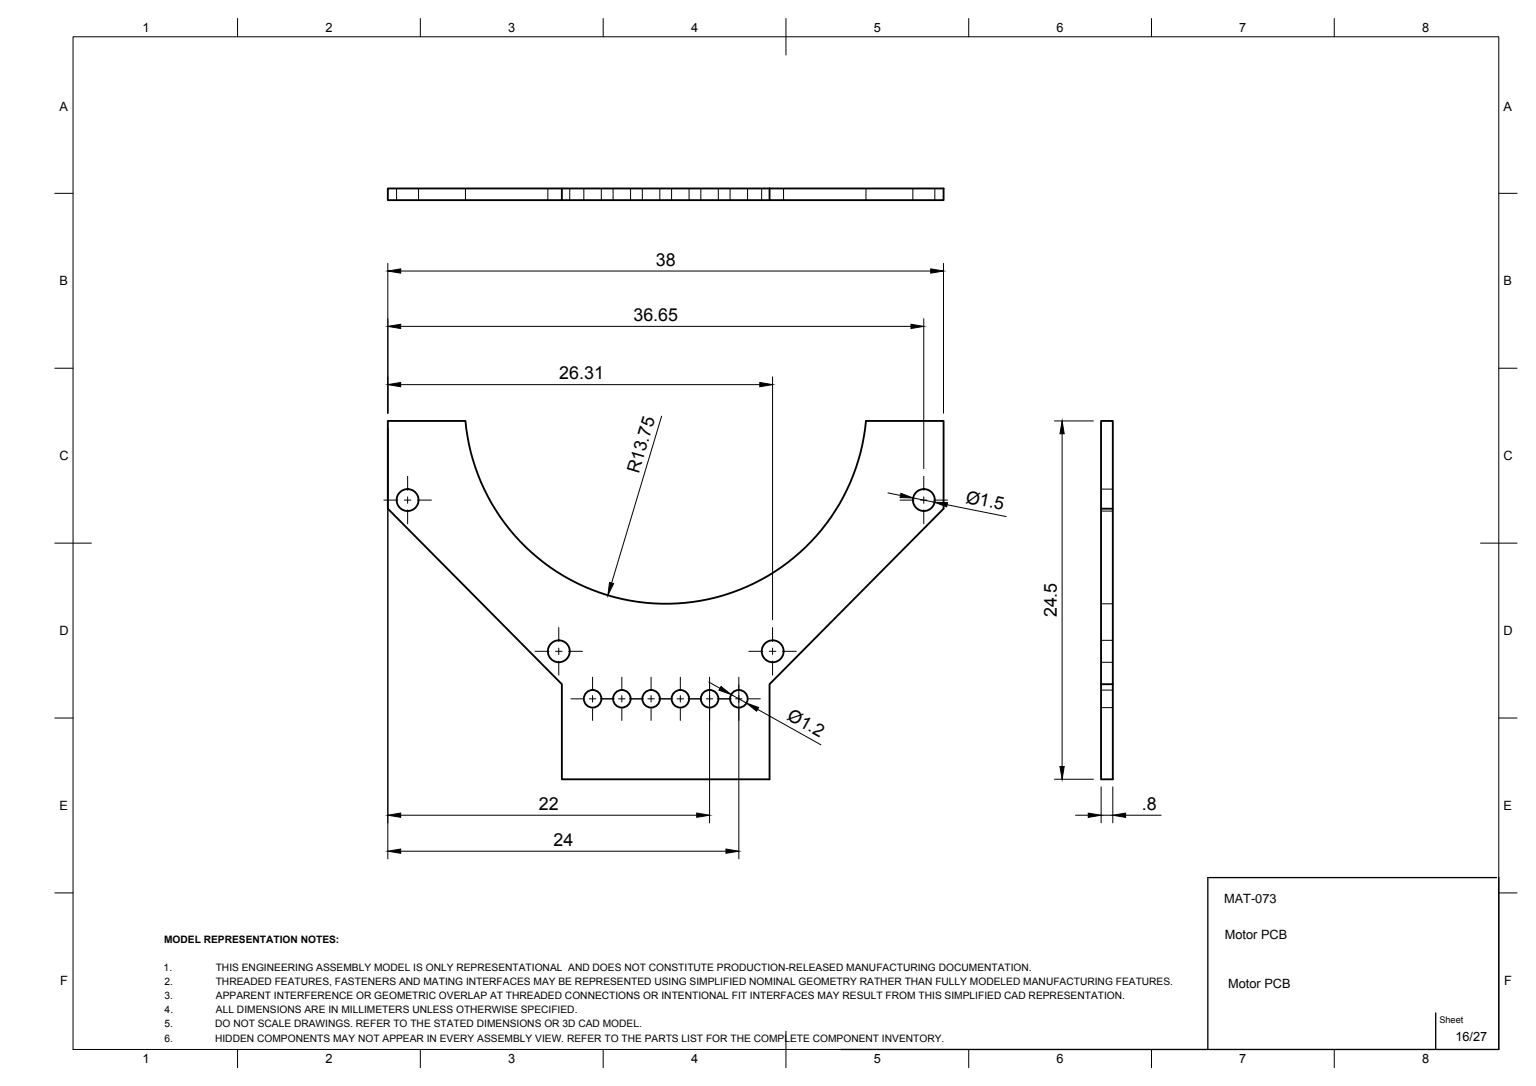
ISO-10303-21;
HEADER;
/* Generated by software containing ST-Developer
 * from STEP Tools, Inc. (www.steptools.com) 
 */

FILE_DESCRIPTION(
/* description */ ('CAx-IF Rec.Pracs.---Representation and Presentation of Product Manufa
cturing Information (PMI)---4.0---2014-10-13'),
/* implementation_level */ '2;1');

FILE_NAME(
/* name */ 'Motor PCB.step',
/* time_stamp */ '2026-10-24T18:52:33-07:00',
/* author */ (''),
/* organization */ (''),
/* preprocessor_version */ 'ST-DEVELOPER v20.2',
/* originating_system */ 'Autodesk Translation Framework v15.17.0.0',
/* authorisation */ '');

FILE_SCHEMA (('AP242_MANAGED_MODEL_BASED_3D_ENGINEERING_MIM_LF { 1 0 10303 442 2 1 4 }'));
ENDSEC;

DATA;
#10=MECHANICAL_DESIGN_GEOMETRIC_PRESENTATION_REPRESENTATION('',(#429),#34876);
#363=SHAPE_REPRESENTATION_RELATIONSHIP('SRR','None',#35000,#396);
#396=ADVANCED_BREP_SHAPE_REPRESENTATION('',(#462),#34858);
#429=STYLED_ITEM('',(#35161),#462);
#462=MANIFOLD_SOLID_BREP('Motor PCB',#19569);
#536=FACE_BOUND('',#6495,.T.);
#537=FACE_BOUND('',#6496,.T.);
#538=FACE_BOUND('',#6497,.T.);
#539=FACE_BOUND('',#6498,.T.);
#540=FACE_BOUND('',#6499,.T.);
#541=FACE_BOUND('',#6500,.T.);
#542=FACE_BOUND('',#6501,.T.);
#543=FACE_BOUND('',#6502,.T.);
#544=FACE_BOUND('',#6503,.T.);
#545=FACE_BOUND('',#6504,.T.);
#546=FACE_BOUND('',#6506,.T.);
#547=FACE_BOUND('',#6507,.T.);
#548=FACE_BOUND('',#6508,.T.);
#549=FACE_BOUND('',#6509,.T.);
#550=FACE_BOUND('',#6510,.T.);
#551=FACE_BOUND('',#6511,.T.);
#552=FACE_BOUND('',#6512,.T.);
#553=FACE_BOUND('',#6513,.T.);
#554=FACE_BOUND('',#6514,.T.);
#555=FACE_BOUND('',#6515,.T.);
#882=PLANE('',#21246);
#883=PLANE('',#21247);
#884=PLANE('',#21248);
#885=PLANE('',#21249);
#886=PLANE('',#21250);
#887=PLANE('',#21251);
#888=PLANE('',#21252);
#889=PLANE('',#21256);
#890=PLANE('',#21257);
#891=PLANE('',#21258);
#892=PLANE('',#21259);
#1947=LINE('',#31950,#3546);
#1948=LINE('',#31956,#3547);
#1949=LINE('',#31962,#3548);
#1950=LINE('',#31968,#3549);
#1951=LINE('',#31974,#3550);
#1952=LINE('',#31980,#3551);
#1953=LINE('',#31986,#3552);
#1954=LINE('',#31992,#3553);
#1955=LINE('',#31998,#3554);
#1956=LINE('',#32004,#3555);
#1957=LINE('',#32009,#3556);
#1958=LINE('',#32011,#3557);
#1959=LINE('',#32013,#3558);
#1960=LINE('',#32014,#3559);
#1961=LINE('',#32017,#3560);
#1962=LINE('',#32019,#3561);
#1963=LINE('',#32020,#3562);
#1964=LINE('',#32024,#3563);
#1965=LINE('',#32026,#3564);
#1966=LINE('',#32028,#3565);
#1967=LINE('',#32029,#3566);
#1968=LINE('',#32031,#3567);
#1969=LINE('',#32032,#3568);
#1970=LINE('',#32036,#3569);
#1971=LINE('',#32038,#3570);
#1972=LINE('',#32040,#3571);
#1973=LINE('',#32041,#3572);
#1974=LINE('',#32044,#3573);
#1975=LINE('',#32046,#3574);
#1976=LINE('',#32047,#3575);
#1977=LINE('',#32049,#3576);
#1978=LINE('',#32050,#3577);
#1979=LINE('',#32056,#3578);
#1980=LINE('',#32059,#3579);
#1981=LINE('',#32061,#3580);
#1982=LINE('',#32062,#3581);
#1983=LINE('',#32064,#3582);
#1984=LINE('',#32065,#3583);
#3546=VECTOR('',#25656,0.00075);
#3547=VECTOR('',#25663,0.00075);
#3548=VECTOR('',#25670,0.00075);
#3549=VECTOR('',#25677,0.00075);
#3550=VECTOR('',#25684,0.0006);
#3551=VECTOR('',#25691,0.0006);
#3552=VECTOR('',#25698,0.0006);
#3553=VECTOR('',#25705,0.0006);
#3554=VECTOR('',#25712,0.0006);
#3555=VECTOR('',#25719,0.0006);
#3556=VECTOR('',#25724,1.);
#3557=VECTOR('',#25725,1.);
#3558=VECTOR('',#25726,1.);
#3559=VECTOR('',#25727,1.);
#3560=VECTOR('',#25730,1.);
#3561=VECTOR('',#25731,1.);
#3562=VECTOR('',#25732,1.);
#3563=VECTOR('',#25735,1.);
#3564=VECTOR('',#25736,1.);
#3565=VECTOR('',#25737,1.);
#3566=VECTOR('',#25738,1.);
#3567=VECTOR('',#25741,1.);
#3568=VECTOR('',#25742,1.);
#3569=VECTOR('',#25745,1.);
#3570=VECTOR('',#25746,1.);
#3571=VECTOR('',#25747,1.);
#3572=VECTOR('',#25748,1.);
#3573=VECTOR('',#25751,1.);
#3574=VECTOR('',#25752,1.);
#3575=VECTOR('',#25753,1.);
#3576=VECTOR('',#25756,1.);
#3577=VECTOR('',#25757,1.);
#3578=VECTOR('',#25764,1.);
#3579=VECTOR('',#25767,1.);
#3580=VECTOR('',#25768,1.);
#3581=VECTOR('',#25769,1.);
#3582=VECTOR('',#25772,1.);
#3583=VECTOR('',#25773,1.);
#4551=CYLINDRICAL_SURFACE('',#21216,0.00075);
#4552=CYLINDRICAL_SURFACE('',#21219,0.00075);
#4553=CYLINDRICAL_SURFACE('',#21222,0.00075);
#4554=CYLINDRICAL_SURFACE('',#21225,0.00075);
#4555=CYLINDRICAL_SURFACE('',#21228,0.0006);
#4556=CYLINDRICAL_SURFACE('',#21231,0.0006);
#4557=CYLINDRICAL_SURFACE('',#21234,0.0006);
#4558=CYLINDRICAL_SURFACE('',#21237,0.0006);
#4559=CYLINDRICAL_SURFACE('',#21240,0.0006);
#4560=CYLINDRICAL_SURFACE('',#21243,0.0006);
#4561=CYLINDRICAL_SURFACE('',#21253,0.01375);
#5373=FACE_OUTER_BOUND('',#6474,.T.);
#5374=FACE_OUTER_BOUND('',#6475,.T.);
#5375=FACE_OUTER_BOUND('',#6476,.T.);
#5376=FACE_OUTER_BOUND('',#6477,.T.);
#5377=FACE_OUTER_BOUND('',#6478,.T.);
#5378=FACE_OUTER_BOUND('',#6479,.T.);
#5379=FACE_OUTER_BOUND('',#6480,.T.);
#5380=FACE_OUTER_BOUND('',#6481,.T.);
#5381=FACE_OUTER_BOUND('',#6482,.T.);
#5382=FACE_OUTER_BOUND('',#6483,.T.);
#5383=FACE_OUTER_BOUND('',#6484,.T.);
#5384=FACE_OUTER_BOUND('',#6485,.T.);
#5385=FACE_OUTER_BOUND('',#6486,.T.);
#5386=FACE_OUTER_BOUND('',#6487,.T.);
#5387=FACE_OUTER_BOUND('',#6488,.T.);
#5388=FACE_OUTER_BOUND('',#6489,.T.);
#5389=FACE_OUTER_BOUND('',#6490,.T.);
#5390=FACE_OUTER_BOUND('',#6491,.T.);
#5391=FACE_OUTER_BOUND('',#6492,.T.);
#5392=FACE_OUTER_BOUND('',#6493,.T.);
#5393=FACE_OUTER_BOUND('',#6494,.T.);
#5394=FACE_OUTER_BOUND('',#6505,.T.);
#6474=EDGE_LOOP('',(#15914,#15915,#15916,#15917));
#6475=EDGE_LOOP('',(#15918,#15919,#15920,#15921));
#6476=EDGE_LOOP('',(#15922,#15923,#15924,#15925));
#6477=EDGE_LOOP('',(#15926,#15927,#15928,#15929));
#6478=EDGE_LOOP('',(#15930,#15931,#15932,#15933));
#6479=EDGE_LOOP('',(#15934,#15935,#15936,#15937));
#6480=EDGE_LOOP('',(#15938,#15939,#15940,#15941));
#6481=EDGE_LOOP('',(#15942,#15943,#15944,#15945));
#6482=EDGE_LOOP('',(#15946,#15947,#15948,#15949));
#6483=EDGE_LOOP('',(#15950,#15951,#15952,#15953));
#6484=EDGE_LOOP('',(#15954,#15955,#15956,#15957));
#6485=EDGE_LOOP('',(#15958,#15959,#15960,#15961));
#6486=EDGE_LOOP('',(#15962,#15963,#15964,#15965));
#6487=EDGE_LOOP('',(#15966,#15967,#15968,#15969));
#6488=EDGE_LOOP('',(#15970,#15971,#15972,#15973));
#6489=EDGE_LOOP('',(#15974,#15975,#15976,#15977));
#6490=EDGE_LOOP('',(#15978,#15979,#15980,#15981));
#6491=EDGE_LOOP('',(#15982,#15983,#15984,#15985));
#6492=EDGE_LOOP('',(#15986,#15987,#15988,#15989));
#6493=EDGE_LOOP('',(#15990,#15991,#15992,#15993));
#6494=EDGE_LOOP('',(#15994,#15995,#15996,#15997,#15998,#15999,#16000,#16001,
#16002,#16003));
#6495=EDGE_LOOP('',(#16004));
#6496=EDGE_LOOP('',(#16005));
#6497=EDGE_LOOP('',(#16006));
#6498=EDGE_LOOP('',(#16007));
#6499=EDGE_LOOP('',(#16008));
#6500=EDGE_LOOP('',(#16009));
#6501=EDGE_LOOP('',(#16010));
#6502=EDGE_LOOP('',(#16011));
#6503=EDGE_LOOP('',(#16012));
#6504=EDGE_LOOP('',(#16013));
#6505=EDGE_LOOP('',(#16014,#16015,#16016,#16017,#16018,#16019,#16020,#16021,
#16022,#16023));
#6506=EDGE_LOOP('',(#16024));
#6507=EDGE_LOOP('',(#16025));
#6508=EDGE_LOOP('',(#16026));
#6509=EDGE_LOOP('',(#16027));
#6510=EDGE_LOOP('',(#16028));
#6511=EDGE_LOOP('',(#16029));
#6512=EDGE_LOOP('',(#16030));
#6513=EDGE_LOOP('',(#16031));
#6514=EDGE_LOOP('',(#16032));
#6515=EDGE_LOOP('',(#16033));
#7549=CIRCLE('',#21217,0.00075000000001);
#7550=CIRCLE('',#21218,0.00075000000001);
#7551=CIRCLE('',#21220,0.00075000000001);
#7552=CIRCLE('',#21221,0.00075000000001);
#7553=CIRCLE('',#21223,0.00075000000001);
#7554=CIRCLE('',#21224,0.00075000000001);
#7555=CIRCLE('',#21226,0.00075000000001);
#7556=CIRCLE('',#21227,0.00075000000001);
#7557=CIRCLE('',#21229,0.00060000000001);
#7558=CIRCLE('',#21230,0.00060000000001);
#7559=CIRCLE('',#21232,0.00060000000001);
#7560=CIRCLE('',#21233,0.00060000000001);
#7561=CIRCLE('',#21235,0.00060000000001);
#7562=CIRCLE('',#21236,0.00060000000001);
#7563=CIRCLE('',#21238,0.00060000000001);
#7564=CIRCLE('',#21239,0.00060000000001);
#7565=CIRCLE('',#21241,0.00060000000001);
#7566=CIRCLE('',#21242,0.00060000000001);
#7567=CIRCLE('',#21244,0.00060000000001);
#7568=CIRCLE('',#21245,0.00060000000001);
#7569=CIRCLE('',#21254,0.01375000000001);
#7570=CIRCLE('',#21255,0.01375000000001);
#9101=VERTEX_POINT('',#31947);
#9102=VERTEX_POINT('',#31949);
#9103=VERTEX_POINT('',#31953);
#9104=VERTEX_POINT('',#31955);
#9105=VERTEX_POINT('',#31959);
#9106=VERTEX_POINT('',#31961);
#9107=VERTEX_POINT('',#31965);
#9108=VERTEX_POINT('',#31967);
#9109=VERTEX_POINT('',#31971);
#9110=VERTEX_POINT('',#31973);
#9111=VERTEX_POINT('',#31977);
#9112=VERTEX_POINT('',#31979);
#9113=VERTEX_POINT('',#31983);
#9114=VERTEX_POINT('',#31985);
#9115=VERTEX_POINT('',#31989);
#9116=VERTEX_POINT('',#31991);
#9117=VERTEX_POINT('',#31995);
#9118=VERTEX_POINT('',#31997);
#9119=VERTEX_POINT('',#32001);
#9120=VERTEX_POINT('',#32003);
#9121=VERTEX_POINT('',#32007);
#9122=VERTEX_POINT('',#32008);
#9123=VERTEX_POINT('',#32010);
#9124=VERTEX_POINT('',#32012);
#9125=VERTEX_POINT('',#32016);
#9126=VERTEX_POINT('',#32018);
#9127=VERTEX_POINT('',#32022);
#9128=VERTEX_POINT('',#32023);
#9129=VERTEX_POINT('',#32025);
#9130=VERTEX_POINT('',#32027);
#9131=VERTEX_POINT('',#32034);
#9132=VERTEX_POINT('',#32035);
#9133=VERTEX_POINT('',#32037);
#9134=VERTEX_POINT('',#32039);
#9135=VERTEX_POINT('',#32043);
#9136=VERTEX_POINT('',#32045);
#9137=VERTEX_POINT('',#32052);
#9138=VERTEX_POINT('',#32054);
#9139=VERTEX_POINT('',#32058);
#9140=VERTEX_POINT('',#32060);
#11515=EDGE_CURVE('',#9101,#9101,#7549,.T.);
#11516=EDGE_CURVE('',#9101,#9102,#1947,.T.);
#11517=EDGE_CURVE('',#9102,#9102,#7550,.T.);
#11518=EDGE_CURVE('',#9103,#9103,#7551,.T.);
#11519=EDGE_CURVE('',#9103,#9104,#1948,.T.);
#11520=EDGE_CURVE('',#9104,#9104,#7552,.T.);
#11521=EDGE_CURVE('',#9105,#9105,#7553,.T.);
#11522=EDGE_CURVE('',#9105,#9106,#1949,.T.);
#11523=EDGE_CURVE('',#9106,#9106,#7554,.T.);
#11524=EDGE_CURVE('',#9107,#9107,#7555,.T.);
#11525=EDGE_CURVE('',#9107,#9108,#1950,.T.);
#11526=EDGE_CURVE('',#9108,#9108,#7556,.T.);
#11527=EDGE_CURVE('',#9109,#9109,#7557,.T.);
#11528=EDGE_CURVE('',#9109,#9110,#1951,.T.);
#11529=EDGE_CURVE('',#9110,#9110,#7558,.T.);
#11530=EDGE_CURVE('',#9111,#9111,#7559,.T.);
#11531=EDGE_CURVE('',#9111,#9112,#1952,.T.);
#11532=EDGE_CURVE('',#9112,#9112,#7560,.T.);
#11533=EDGE_CURVE('',#9113,#9113,#7561,.T.);
#11534=EDGE_CURVE('',#9113,#9114,#1953,.T.);
#11535=EDGE_CURVE('',#9114,#9114,#7562,.T.);
#11536=EDGE_CURVE('',#9115,#9115,#7563,.T.);
#11537=EDGE_CURVE('',#9115,#9116,#1954,.T.);
#11538=EDGE_CURVE('',#9116,#9116,#7564,.T.);
#11539=EDGE_CURVE('',#9117,#9117,#7565,.T.);
#11540=EDGE_CURVE('',#9117,#9118,#1955,.T.);
#11541=EDGE_CURVE('',#9118,#9118,#7566,.T.);
#11542=EDGE_CURVE('',#9119,#9119,#7567,.T.);
#11543=EDGE_CURVE('',#9119,#9120,#1956,.T.);
#11544=EDGE_CURVE('',#9120,#9120,#7568,.T.);
#11545=EDGE_CURVE('',#9121,#9122,#1957,.T.);
#11546=EDGE_CURVE('',#9121,#9123,#1958,.T.);
#11547=EDGE_CURVE('',#9123,#9124,#1959,.T.);
#11548=EDGE_CURVE('',#9122,#9124,#1960,.T.);
#11549=EDGE_CURVE('',#9125,#9121,#1961,.T.);
#11550=EDGE_CURVE('',#9125,#9126,#1962,.T.);
#11551=EDGE_CURVE('',#9126,#9123,#1963,.T.);
#11552=EDGE_CURVE('',#9127,#9128,#1964,.T.);
#11553=EDGE_CURVE('',#9127,#9129,#1965,.T.);
#11554=EDGE_CURVE('',#9129,#9130,#1966,.T.);
#11555=EDGE_CURVE('',#9128,#9130,#1967,.T.);
#11556=EDGE_CURVE('',#9122,#9127,#1968,.T.);
#11557=EDGE_CURVE('',#9124,#9129,#1969,.T.);
#11558=EDGE_CURVE('',#9131,#9132,#1970,.T.);
#11559=EDGE_CURVE('',#9132,#9133,#1971,.T.);
#11560=EDGE_CURVE('',#9134,#9133,#1972,.T.);
#11561=EDGE_CURVE('',#9131,#9134,#1973,.T.);
#11562=EDGE_CURVE('',#9135,#9131,#1974,.T.);
#11563=EDGE_CURVE('',#9136,#9134,#1975,.T.);
#11564=EDGE_CURVE('',#9135,#9136,#1976,.T.);
#11565=EDGE_CURVE('',#9135,#9125,#1977,.T.);
#11566=EDGE_CURVE('',#9136,#9126,#1978,.T.);
#11567=EDGE_CURVE('',#9137,#9128,#7569,.T.);
#11568=EDGE_CURVE('',#9138,#9130,#7570,.T.);
#11569=EDGE_CURVE('',#9137,#9138,#1979,.T.);
#11570=EDGE_CURVE('',#9139,#9137,#1980,.T.);
#11571=EDGE_CURVE('',#9140,#9138,#1981,.T.);
#11572=EDGE_CURVE('',#9139,#9140,#1982,.T.);
#11573=EDGE_CURVE('',#9132,#9139,#1983,.T.);
#11574=EDGE_CURVE('',#9133,#9140,#1984,.T.);
#15914=ORIENTED_EDGE('',*,*,#11515,.F.);
#15915=ORIENTED_EDGE('',*,*,#11516,.T.);
#15916=ORIENTED_EDGE('',*,*,#11517,.F.);
#15917=ORIENTED_EDGE('',*,*,#11516,.F.);
#15918=ORIENTED_EDGE('',*,*,#11518,.F.);
#15919=ORIENTED_EDGE('',*,*,#11519,.T.);
#15920=ORIENTED_EDGE('',*,*,#11520,.F.);
#15921=ORIENTED_EDGE('',*,*,#11519,.F.);
#15922=ORIENTED_EDGE('',*,*,#11521,.F.);
#15923=ORIENTED_EDGE('',*,*,#11522,.T.);
#15924=ORIENTED_EDGE('',*,*,#11523,.F.);
#15925=ORIENTED_EDGE('',*,*,#11522,.F.);
#15926=ORIENTED_EDGE('',*,*,#11524,.F.);
#15927=ORIENTED_EDGE('',*,*,#11525,.T.);
#15928=ORIENTED_EDGE('',*,*,#11526,.F.);
#15929=ORIENTED_EDGE('',*,*,#11525,.F.);
#15930=ORIENTED_EDGE('',*,*,#11527,.F.);
#15931=ORIENTED_EDGE('',*,*,#11528,.T.);
#15932=ORIENTED_EDGE('',*,*,#11529,.F.);
#15933=ORIENTED_EDGE('',*,*,#11528,.F.);
#15934=ORIENTED_EDGE('',*,*,#11530,.F.);
#15935=ORIENTED_EDGE('',*,*,#11531,.T.);
#15936=ORIENTED_EDGE('',*,*,#11532,.F.);
#15937=ORIENTED_EDGE('',*,*,#11531,.F.);
#15938=ORIENTED_EDGE('',*,*,#11533,.F.);
#15939=ORIENTED_EDGE('',*,*,#11534,.T.);
#15940=ORIENTED_EDGE('',*,*,#11535,.F.);
#15941=ORIENTED_EDGE('',*,*,#11534,.F.);
#15942=ORIENTED_EDGE('',*,*,#11536,.F.);
#15943=ORIENTED_EDGE('',*,*,#11537,.T.);
#15944=ORIENTED_EDGE('',*,*,#11538,.F.);
#15945=ORIENTED_EDGE('',*,*,#11537,.F.);
#15946=ORIENTED_EDGE('',*,*,#11539,.F.);
#15947=ORIENTED_EDGE('',*,*,#11540,.T.);
#15948=ORIENTED_EDGE('',*,*,#11541,.F.);
#15949=ORIENTED_EDGE('',*,*,#11540,.F.);
#15950=ORIENTED_EDGE('',*,*,#11542,.F.);
#15951=ORIENTED_EDGE('',*,*,#11543,.T.);
#15952=ORIENTED_EDGE('',*,*,#11544,.F.);
#15953=ORIENTED_EDGE('',*,*,#11543,.F.);
#15954=ORIENTED_EDGE('',*,*,#11545,.F.);
#15955=ORIENTED_EDGE('',*,*,#11546,.T.);
#15956=ORIENTED_EDGE('',*,*,#11547,.T.);
#15957=ORIENTED_EDGE('',*,*,#11548,.F.);
#15958=ORIENTED_EDGE('',*,*,#11549,.F.);
#15959=ORIENTED_EDGE('',*,*,#11550,.T.);
#15960=ORIENTED_EDGE('',*,*,#11551,.T.);
#15961=ORIENTED_EDGE('',*,*,#11546,.F.);
#15962=ORIENTED_EDGE('',*,*,#11552,.F.);
#15963=ORIENTED_EDGE('',*,*,#11553,.T.);
#15964=ORIENTED_EDGE('',*,*,#11554,.T.);
#15965=ORIENTED_EDGE('',*,*,#11555,.F.);
#15966=ORIENTED_EDGE('',*,*,#11556,.F.);
#15967=ORIENTED_EDGE('',*,*,#11548,.T.);
#15968=ORIENTED_EDGE('',*,*,#11557,.T.);
#15969=ORIENTED_EDGE('',*,*,#11553,.F.);
#15970=ORIENTED_EDGE('',*,*,#11558,.T.);
#15971=ORIENTED_EDGE('',*,*,#11559,.T.);
#15972=ORIENTED_EDGE('',*,*,#11560,.F.);
#15973=ORIENTED_EDGE('',*,*,#11561,.F.);
#15974=ORIENTED_EDGE('',*,*,#11562,.T.);
#15975=ORIENTED_EDGE('',*,*,#11561,.T.);
#15976=ORIENTED_EDGE('',*,*,#11563,.F.);
#15977=ORIENTED_EDGE('',*,*,#11564,.F.);
#15978=ORIENTED_EDGE('',*,*,#11565,.F.);
#15979=ORIENTED_EDGE('',*,*,#11564,.T.);
#15980=ORIENTED_EDGE('',*,*,#11566,.T.);
#15981=ORIENTED_EDGE('',*,*,#11550,.F.);
#15982=ORIENTED_EDGE('',*,*,#11567,.T.);
#15983=ORIENTED_EDGE('',*,*,#11555,.T.);
#15984=ORIENTED_EDGE('',*,*,#11568,.F.);
#15985=ORIENTED_EDGE('',*,*,#11569,.F.);
#15986=ORIENTED_EDGE('',*,*,#11570,.T.);
#15987=ORIENTED_EDGE('',*,*,#11569,.T.);
#15988=ORIENTED_EDGE('',*,*,#11571,.F.);
#15989=ORIENTED_EDGE('',*,*,#11572,.F.);
#15990=ORIENTED_EDGE('',*,*,#11573,.T.);
#15991=ORIENTED_EDGE('',*,*,#11572,.T.);
#15992=ORIENTED_EDGE('',*,*,#11574,.F.);
#15993=ORIENTED_EDGE('',*,*,#11559,.F.);
#15994=ORIENTED_EDGE('',*,*,#11574,.T.);
#15995=ORIENTED_EDGE('',*,*,#11571,.T.);
#15996=ORIENTED_EDGE('',*,*,#11568,.T.);
#15997=ORIENTED_EDGE('',*,*,#11554,.F.);
#15998=ORIENTED_EDGE('',*,*,#11557,.F.);
#15999=ORIENTED_EDGE('',*,*,#11547,.F.);
#16000=ORIENTED_EDGE('',*,*,#11551,.F.);
#16001=ORIENTED_EDGE('',*,*,#11566,.F.);
#16002=ORIENTED_EDGE('',*,*,#11563,.T.);
#16003=ORIENTED_EDGE('',*,*,#11560,.T.);
#16004=ORIENTED_EDGE('',*,*,#11517,.T.);
#16005=ORIENTED_EDGE('',*,*,#11520,.T.);
#16006=ORIENTED_EDGE('',*,*,#11523,.T.);
#16007=ORIENTED_EDGE('',*,*,#11526,.T.);
#16008=ORIENTED_EDGE('',*,*,#11529,.T.);
#16009=ORIENTED_EDGE('',*,*,#11532,.T.);
#16010=ORIENTED_EDGE('',*,*,#11535,.T.);
#16011=ORIENTED_EDGE('',*,*,#11538,.T.);
#16012=ORIENTED_EDGE('',*,*,#11541,.T.);
#16013=ORIENTED_EDGE('',*,*,#11544,.T.);
#16014=ORIENTED_EDGE('',*,*,#11573,.F.);
#16015=ORIENTED_EDGE('',*,*,#11558,.F.);
#16016=ORIENTED_EDGE('',*,*,#11562,.F.);
#16017=ORIENTED_EDGE('',*,*,#11565,.T.);
#16018=ORIENTED_EDGE('',*,*,#11549,.T.);
#16019=ORIENTED_EDGE('',*,*,#11545,.T.);
#16020=ORIENTED_EDGE('',*,*,#11556,.T.);
#16021=ORIENTED_EDGE('',*,*,#11552,.T.);
#16022=ORIENTED_EDGE('',*,*,#11567,.F.);
#16023=ORIENTED_EDGE('',*,*,#11570,.F.);
#16024=ORIENTED_EDGE('',*,*,#11515,.T.);
#16025=ORIENTED_EDGE('',*,*,#11518,.T.);
#16026=ORIENTED_EDGE('',*,*,#11521,.T.);
#16027=ORIENTED_EDGE('',*,*,#11524,.T.);
#16028=ORIENTED_EDGE('',*,*,#11527,.T.);
#16029=ORIENTED_EDGE('',*,*,#11530,.T.);
#16030=ORIENTED_EDGE('',*,*,#11533,.T.);
#16031=ORIENTED_EDGE('',*,*,#11536,.T.);
#16032=ORIENTED_EDGE('',*,*,#11539,.T.);
#16033=ORIENTED_EDGE('',*,*,#11542,.T.);
#19089=ADVANCED_FACE('',(#5373),#4551,.F.);
#19090=ADVANCED_FACE('',(#5374),#4552,.F.);
#19091=ADVANCED_FACE('',(#5375),#4553,.F.);
#19092=ADVANCED_FACE('',(#5376),#4554,.F.);
#19093=ADVANCED_FACE('',(#5377),#4555,.F.);
#19094=ADVANCED_FACE('',(#5378),#4556,.F.);
#19095=ADVANCED_FACE('',(#5379),#4557,.F.);
#19096=ADVANCED_FACE('',(#5380),#4558,.F.);
#19097=ADVANCED_FACE('',(#5381),#4559,.F.);
#19098=ADVANCED_FACE('',(#5382),#4560,.F.);
#19099=ADVANCED_FACE('',(#5383),#882,.F.);
#19100=ADVANCED_FACE('',(#5384),#883,.F.);
#19101=ADVANCED_FACE('',(#5385),#884,.F.);
#19102=ADVANCED_FACE('',(#5386),#885,.F.);
#19103=ADVANCED_FACE('',(#5387),#886,.T.);
#19104=ADVANCED_FACE('',(#5388),#887,.T.);
#19105=ADVANCED_FACE('',(#5389),#888,.T.);
#19106=ADVANCED_FACE('',(#5390),#4561,.F.);
#19107=ADVANCED_FACE('',(#5391),#889,.T.);
#19108=ADVANCED_FACE('',(#5392),#890,.T.);
#19109=ADVANCED_FACE('',(#5393,#536,#537,#538,#539,#540,#541,#542,#543,
#544,#545),#891,.T.);
#19110=ADVANCED_FACE('',(#5394,#546,#547,#548,#549,#550,#551,#552,#553,
#554,#555),#892,.F.);
#19569=CLOSED_SHELL('',(#19089,#19090,#19091,#19092,#19093,#19094,#19095,
#19096,#19097,#19098,#19099,#19100,#19101,#19102,#19103,#19104,#19105,#19106,
#19107,#19108,#19109,#19110));
#21215=AXIS2_PLACEMENT_3D('',#31945,#25650,#25651);
#21216=AXIS2_PLACEMENT_3D('',#31946,#25652,#25653);
#21217=AXIS2_PLACEMENT_3D('',#31948,#25654,#25655);
#21218=AXIS2_PLACEMENT_3D('',#31951,#25657,#25658);
#21219=AXIS2_PLACEMENT_3D('',#31952,#25659,#25660);
#21220=AXIS2_PLACEMENT_3D('',#31954,#25661,#25662);
#21221=AXIS2_PLACEMENT_3D('',#31957,#25664,#25665);
#21222=AXIS2_PLACEMENT_3D('',#31958,#25666,#25667);
#21223=AXIS2_PLACEMENT_3D('',#31960,#25668,#25669);
#21224=AXIS2_PLACEMENT_3D('',#31963,#25671,#25672);
#21225=AXIS2_PLACEMENT_3D('',#31964,#25673,#25674);
#21226=AXIS2_PLACEMENT_3D('',#31966,#25675,#25676);
#21227=AXIS2_PLACEMENT_3D('',#31969,#25678,#25679);
#21228=AXIS2_PLACEMENT_3D('',#31970,#25680,#25681);
#21229=AXIS2_PLACEMENT_3D('',#31972,#25682,#25683);
#21230=AXIS2_PLACEMENT_3D('',#31975,#25685,#25686);
#21231=AXIS2_PLACEMENT_3D('',#31976,#25687,#25688);
#21232=AXIS2_PLACEMENT_3D('',#31978,#25689,#25690);
#21233=AXIS2_PLACEMENT_3D('',#31981,#25692,#25693);
#21234=AXIS2_PLACEMENT_3D('',#31982,#25694,#25695);
#21235=AXIS2_PLACEMENT_3D('',#31984,#25696,#25697);
#21236=AXIS2_PLACEMENT_3D('',#31987,#25699,#25700);
#21237=AXIS2_PLACEMENT_3D('',#31988,#25701,#25702);
#21238=AXIS2_PLACEMENT_3D('',#31990,#25703,#25704);
#21239=AXIS2_PLACEMENT_3D('',#31993,#25706,#25707);
#21240=AXIS2_PLACEMENT_3D('',#31994,#25708,#25709);
#21241=AXIS2_PLACEMENT_3D('',#31996,#25710,#25711);
#21242=AXIS2_PLACEMENT_3D('',#31999,#25713,#25714);
#21243=AXIS2_PLACEMENT_3D('',#32000,#25715,#25716);
#21244=AXIS2_PLACEMENT_3D('',#32002,#25717,#25718);
#21245=AXIS2_PLACEMENT_3D('',#32005,#25720,#25721);
#21246=AXIS2_PLACEMENT_3D('',#32006,#25722,#25723);
#21247=AXIS2_PLACEMENT_3D('',#32015,#25728,#25729);
#21248=AXIS2_PLACEMENT_3D('',#32021,#25733,#25734);
#21249=AXIS2_PLACEMENT_3D('',#32030,#25739,#25740);
#21250=AXIS2_PLACEMENT_3D('',#32033,#25743,#25744);
#21251=AXIS2_PLACEMENT_3D('',#32042,#25749,#25750);
#21252=AXIS2_PLACEMENT_3D('',#32048,#25754,#25755);
#21253=AXIS2_PLACEMENT_3D('',#32051,#25758,#25759);
#21254=AXIS2_PLACEMENT_3D('',#32053,#25760,#25761);
#21255=AXIS2_PLACEMENT_3D('',#32055,#25762,#25763);
#21256=AXIS2_PLACEMENT_3D('',#32057,#25765,#25766);
#21257=AXIS2_PLACEMENT_3D('',#32063,#25770,#25771);
#21258=AXIS2_PLACEMENT_3D('',#32066,#25774,#25775);
#21259=AXIS2_PLACEMENT_3D('',#32067,#25776,#25777);
#25650=DIRECTION('axis',(0.,0.,1.));
#25651=DIRECTION('refdir',(1.,0.,0.));
#25652=DIRECTION('center_axis',(4.57029560239561E-17,1.,8.81733986229836E-18));
#25653=DIRECTION('ref_axis',(4.44089209850056E-15,-8.81733986229857E-18,
1.));
#25654=DIRECTION('center_axis',(4.57029560239561E-17,1.,8.81733986229836E-18));
#25655=DIRECTION('ref_axis',(4.44089209850056E-15,-8.81733986229857E-18,
1.));
#25656=DIRECTION('',(4.57029560239561E-17,1.,8.81733986229836E-18));
#25657=DIRECTION('center_axis',(-4.57029560239561E-17,-1.,-8.81733986229836E-18));
#25658=DIRECTION('ref_axis',(4.44089209850056E-15,-8.81733986229857E-18,
1.));
#25659=DIRECTION('center_axis',(4.57029560239561E-17,1.,8.81733986229836E-18));
#25660=DIRECTION('ref_axis',(4.44089209850056E-15,-8.81733986229857E-18,
1.));
#25661=DIRECTION('center_axis',(4.57029560239561E-17,1.,8.81733986229836E-18));
#25662=DIRECTION('ref_axis',(4.44089209850056E-15,-8.81733986229857E-18,
1.));
#25663=DIRECTION('',(4.57029560239561E-17,1.,8.81733986229836E-18));
#25664=DIRECTION('center_axis',(-4.57029560239561E-17,-1.,-8.81733986229836E-18));
#25665=DIRECTION('ref_axis',(4.44089209850056E-15,-8.81733986229857E-18,
1.));
#25666=DIRECTION('center_axis',(4.57029560239561E-17,1.,8.81733986229836E-18));
#25667=DIRECTION('ref_axis',(4.44089209850056E-15,-8.81733986229857E-18,
1.));
#25668=DIRECTION('center_axis',(4.57029560239561E-17,1.,8.81733986229836E-18));
#25669=DIRECTION('ref_axis',(4.44089209850056E-15,-8.81733986229857E-18,
1.));
#25670=DIRECTION('',(4.57029560239561E-17,1.,8.81733986229836E-18));
#25671=DIRECTION('center_axis',(-4.57029560239561E-17,-1.,-8.81733986229836E-18));
#25672=DIRECTION('ref_axis',(4.44089209850056E-15,-8.81733986229857E-18,
1.));
#25673=DIRECTION('center_axis',(4.57029560239561E-17,1.,8.81733986229836E-18));
#25674=DIRECTION('ref_axis',(4.44089209850056E-15,-8.81733986229857E-18,
1.));
#25675=DIRECTION('center_axis',(4.57029560239561E-17,1.,8.81733986229836E-18));
#25676=DIRECTION('ref_axis',(4.44089209850056E-15,-8.81733986229857E-18,
1.));
#25677=DIRECTION('',(4.57029560239561E-17,1.,8.81733986229836E-18));
#25678=DIRECTION('center_axis',(-4.57029560239561E-17,-1.,-8.81733986229836E-18));
#25679=DIRECTION('ref_axis',(4.44089209850056E-15,-8.81733986229857E-18,
1.));
#25680=DIRECTION('center_axis',(4.57029560239561E-17,1.,8.81733986229836E-18));
#25681=DIRECTION('ref_axis',(4.44089209850056E-15,-8.81733986229857E-18,
1.));
#25682=DIRECTION('center_axis',(4.57029560239561E-17,1.,8.81733986229836E-18));
#25683=DIRECTION('ref_axis',(4.44089209850056E-15,-8.81733986229856E-18,
1.));
#25684=DIRECTION('',(4.57029560239561E-17,1.,8.81733986229836E-18));
#25685=DIRECTION('center_axis',(-4.57029560239561E-17,-1.,-8.81733986229836E-18));
#25686=DIRECTION('ref_axis',(4.44089209850056E-15,-8.81733986229856E-18,
1.));
#25687=DIRECTION('center_axis',(4.57029560239561E-17,1.,8.81733986229836E-18));
#25688=DIRECTION('ref_axis',(4.44089209850056E-15,-8.81733986229857E-18,
1.));
#25689=DIRECTION('center_axis',(4.57029560239561E-17,1.,8.81733986229836E-18));
#25690=DIRECTION('ref_axis',(4.44089209850056E-15,-8.81733986229856E-18,
1.));
#25691=DIRECTION('',(4.57029560239561E-17,1.,8.81733986229836E-18));
#25692=DIRECTION('center_axis',(-4.57029560239561E-17,-1.,-8.81733986229836E-18));
#25693=DIRECTION('ref_axis',(4.44089209850056E-15,-8.81733986229856E-18,
1.));
#25694=DIRECTION('center_axis',(4.57029560239561E-17,1.,8.81733986229836E-18));
#25695=DIRECTION('ref_axis',(4.44089209850056E-15,-8.81733986229857E-18,
1.));
#25696=DIRECTION('center_axis',(4.57029560239561E-17,1.,8.81733986229836E-18));
#25697=DIRECTION('ref_axis',(4.44089209850056E-15,-8.81733986229856E-18,
1.));
#25698=DIRECTION('',(4.57029560239561E-17,1.,8.81733986229836E-18));
#25699=DIRECTION('center_axis',(-4.57029560239561E-17,-1.,-8.81733986229836E-18));
#25700=DIRECTION('ref_axis',(4.44089209850056E-15,-8.81733986229856E-18,
1.));
#25701=DIRECTION('center_axis',(4.57029560239561E-17,1.,8.81733986229836E-18));
#25702=DIRECTION('ref_axis',(4.44089209850056E-15,-8.81733986229857E-18,
1.));
#25703=DIRECTION('center_axis',(4.57029560239561E-17,1.,8.81733986229836E-18));
#25704=DIRECTION('ref_axis',(4.44089209850056E-15,-8.81733986229856E-18,
1.));
#25705=DIRECTION('',(4.57029560239561E-17,1.,8.81733986229836E-18));
#25706=DIRECTION('center_axis',(-4.57029560239561E-17,-1.,-8.81733986229836E-18));
#25707=DIRECTION('ref_axis',(4.44089209850056E-15,-8.81733986229856E-18,
1.));
#25708=DIRECTION('center_axis',(4.57029560239561E-17,1.,8.81733986229836E-18));
#25709=DIRECTION('ref_axis',(4.44089209850056E-15,-8.81733986229857E-18,
1.));
#25710=DIRECTION('center_axis',(4.57029560239561E-17,1.,8.81733986229836E-18));
#25711=DIRECTION('ref_axis',(4.44089209850056E-15,-8.81733986229856E-18,
1.));
#25712=DIRECTION('',(4.57029560239561E-17,1.,8.81733986229836E-18));
#25713=DIRECTION('center_axis',(-4.57029560239561E-17,-1.,-8.81733986229836E-18));
#25714=DIRECTION('ref_axis',(4.44089209850056E-15,-8.81733986229856E-18,
1.));
#25715=DIRECTION('center_axis',(4.57029560239561E-17,1.,8.81733986229836E-18));
#25716=DIRECTION('ref_axis',(4.44089209850056E-15,-8.81733986229857E-18,
1.));
#25717=DIRECTION('center_axis',(4.57029560239561E-17,1.,8.81733986229836E-18));
#25718=DIRECTION('ref_axis',(4.44089209850056E-15,-8.81733986229856E-18,
1.));
#25719=DIRECTION('',(4.57029560239561E-17,1.,8.81733986229836E-18));
#25720=DIRECTION('center_axis',(-4.57029560239561E-17,-1.,-8.81733986229836E-18));
#25721=DIRECTION('ref_axis',(4.44089209850056E-15,-8.81733986229856E-18,
1.));
#25722=DIRECTION('center_axis',(-0.704142011834323,3.84422044398024E-17,
-0.71005917159763));
#25723=DIRECTION('ref_axis',(4.57029560239561E-17,1.,8.81733986229838E-18));
#25724=DIRECTION('',(-0.710059171597626,2.62431436642672E-17,0.704142011834327));
#25725=DIRECTION('',(4.57029560239561E-17,1.,8.81733986229836E-18));
#25726=DIRECTION('',(-0.710059171597626,2.62431436642672E-17,0.704142011834327));
#25727=DIRECTION('',(4.57029560239561E-17,1.,8.81733986229836E-18));
#25728=DIRECTION('center_axis',(-4.69798701365815E-15,8.81733986229857E-18,
-1.));
#25729=DIRECTION('ref_axis',(4.57029560239561E-17,1.,8.81733986229836E-18));
#25730=DIRECTION('',(-1.,4.57029560239473E-17,1.00469798701266E-12));
#25731=DIRECTION('',(4.57029560239561E-17,1.,8.81733986229836E-18));
#25732=DIRECTION('',(-1.,4.57029560239473E-17,1.00469798701266E-12));
#25733=DIRECTION('center_axis',(1.,-4.57029560239561E-17,-4.42423575072469E-15));
#25734=DIRECTION('ref_axis',(-4.57029560239561E-17,-1.,-8.81733986229836E-18));
#25735=DIRECTION('',(9.95575764248275E-13,8.81733986225286E-18,-1.));
#25736=DIRECTION('',(4.57029560239561E-17,1.,8.81733986229836E-18));
#25737=DIRECTION('',(9.95575764248275E-13,8.81733986225286E-18,-1.));
#25738=DIRECTION('',(4.57029560239561E-17,1.,8.81733986229836E-18));
#25739=DIRECTION('center_axis',(-4.49871621436646E-15,8.81733986229856E-18,
-1.));
#25740=DIRECTION('ref_axis',(4.57029560239561E-17,1.,8.81733986229835E-18));
#25741=DIRECTION('',(-1.,4.57029560239473E-17,1.00449871621337E-12));
#25742=DIRECTION('',(-1.,4.57029560239473E-17,1.00449871621337E-12));
#25743=DIRECTION('center_axis',(0.704142011834316,-2.59205383631653E-17,
-0.710059171597636));
#25744=DIRECTION('ref_axis',(-0.710059171597636,3.86604625235991E-17,-0.704142011834316));
#25745=DIRECTION('',(-0.710059171597632,3.8660462523599E-17,-0.704142011834321));
#25746=DIRECTION('',(4.57029560239561E-17,1.,8.81733986229836E-18));
#25747=DIRECTION('',(-0.710059171597632,3.8660462523599E-17,-0.704142011834321));
#25748=DIRECTION('',(4.57029560239561E-17,1.,8.81733986229836E-18));
#25749=DIRECTION('center_axis',(-4.61169564075059E-15,8.81733986229857E-18,
-1.));
#25750=DIRECTION('ref_axis',(4.57029560239561E-17,1.,8.81733986229836E-18));
#25751=DIRECTION('',(-1.,4.57029560239473E-17,1.00461169563975E-12));
#25752=DIRECTION('',(-1.,4.57029560239473E-17,1.00461169563975E-12));
#25753=DIRECTION('',(4.57029560239561E-17,1.,8.81733986229836E-18));
#25754=DIRECTION('center_axis',(1.,-4.57029560239561E-17,-4.44089209850056E-15));
#25755=DIRECTION('ref_axis',(-4.57029560239561E-17,-1.,-8.81733986229836E-18));
#25756=DIRECTION('',(1.00486879055491E-12,-8.81733986234428E-18,1.));
#25757=DIRECTION('',(1.00486879055491E-12,-8.81733986234428E-18,1.));
#25758=DIRECTION('center_axis',(4.57029560239561E-17,1.,8.81733986229836E-18));
#25759=DIRECTION('ref_axis',(4.44089209850056E-15,-8.81733986229856E-18,
1.));
#25760=DIRECTION('center_axis',(-4.57029560239561E-17,-1.,-8.81733986229836E-18));
#25761=DIRECTION('ref_axis',(4.44089209850056E-15,-8.81733986229856E-18,
1.));
#25762=DIRECTION('center_axis',(-4.57029560239561E-17,-1.,-8.81733986229836E-18));
#25763=DIRECTION('ref_axis',(4.44089209850056E-15,-8.81733986229856E-18,
1.));
#25764=DIRECTION('',(4.57029560239561E-17,1.,8.81733986229836E-18));
#25765=DIRECTION('center_axis',(-1.,4.57029560239563E-17,4.44089209850056E-15));
#25766=DIRECTION('ref_axis',(4.44089209850056E-15,-4.5337214504578E-16,
1.));
#25767=DIRECTION('',(1.00488544690268E-12,-8.81733986234428E-18,1.));
#25768=DIRECTION('',(1.00488544690268E-12,-8.81733986234428E-18,1.));
#25769=DIRECTION('',(4.57029560239561E-17,1.,8.81733986229836E-18));
#25770=DIRECTION('center_axis',(-4.81096644004228E-15,8.81733986229858E-18,
-1.));
#25771=DIRECTION('ref_axis',(4.57029560239561E-17,1.,8.81733986229836E-18));
#25772=DIRECTION('',(-1.,4.57029560239473E-17,1.00481096643904E-12));
#25773=DIRECTION('',(-1.,4.57029560239473E-17,1.00481096643904E-12));
#25774=DIRECTION('center_axis',(4.57029560239561E-17,1.,8.81733986229836E-18));
#25775=DIRECTION('ref_axis',(4.44089209850056E-15,-8.81733986229856E-18,
1.));
#25776=DIRECTION('center_axis',(4.57029560239561E-17,1.,8.81733986229836E-18));
#25777=DIRECTION('ref_axis',(4.44089209850056E-15,-8.81733986229856E-18,
1.));
#31945=CARTESIAN_POINT('',(0.,0.,0.));
#31946=CARTESIAN_POINT('Origin',(0.01765,-0.03005,-0.00731086937588517));
#31947=CARTESIAN_POINT('',(0.01765,-0.03005,-0.00806086937588517));
#31948=CARTESIAN_POINT('Origin',(0.01765000000001,-0.03005,-0.00731086937589517));
#31949=CARTESIAN_POINT('',(0.01765,-0.02924999999999,-0.00806086937588517));
#31950=CARTESIAN_POINT('',(0.01765,-0.03005,-0.00806086937588517));
#31951=CARTESIAN_POINT('Origin',(0.01765000000001,-0.02924999999999,-0.00731086937589517));
#31952=CARTESIAN_POINT('Origin',(0.01765,-0.03005,0.0073108693758851));
#31953=CARTESIAN_POINT('',(0.01765,-0.03005,0.0065608693758851));
#31954=CARTESIAN_POINT('Origin',(0.0176500000000099,-0.03005,0.0073108693758951));
#31955=CARTESIAN_POINT('',(0.01765,-0.02924999999999,0.0065608693758851));
#31956=CARTESIAN_POINT('',(0.01765,-0.03005,0.0065608693758851));
#31957=CARTESIAN_POINT('Origin',(0.0176500000000099,-0.02924999999999,0.0073108693758951));
#31958=CARTESIAN_POINT('Origin',(0.00731086937588504,-0.03005,-0.01765));
#31959=CARTESIAN_POINT('',(0.00731086937588504,-0.03005,-0.0184));
#31960=CARTESIAN_POINT('Origin',(0.00731086937589504,-0.03005,-0.0176500000000101));
#31961=CARTESIAN_POINT('',(0.00731086937588504,-0.02924999999999,-0.0184));
#31962=CARTESIAN_POINT('',(0.00731086937588504,-0.03005,-0.0184));
#31963=CARTESIAN_POINT('Origin',(0.00731086937589504,-0.02924999999999,
-0.0176500000000101));
#31964=CARTESIAN_POINT('Origin',(0.00731086937588512,-0.03005,0.01765));
#31965=CARTESIAN_POINT('',(0.00731086937588512,-0.03005,0.0169));
#31966=CARTESIAN_POINT('Origin',(0.00731086937589512,-0.03005,0.0176500000000099));
#31967=CARTESIAN_POINT('',(0.00731086937588512,-0.02924999999999,0.0169));
#31968=CARTESIAN_POINT('',(0.00731086937588512,-0.03005,0.0169));
#31969=CARTESIAN_POINT('Origin',(0.00731086937589512,-0.02924999999999,
0.0176500000000099));
#31970=CARTESIAN_POINT('Origin',(0.0209,-0.0744704599711237,0.005));
#31971=CARTESIAN_POINT('',(0.0209,-0.03005,0.0044));
#31972=CARTESIAN_POINT('Origin',(0.02090000000001,-0.03005,0.00500000000001));
#31973=CARTESIAN_POINT('',(0.0209,-0.02924999999999,0.0044));
#31974=CARTESIAN_POINT('',(0.0209,-0.0744704599711237,0.0044));
#31975=CARTESIAN_POINT('Origin',(0.02090000000001,-0.02924999999999,0.00500000000001));
#31976=CARTESIAN_POINT('Origin',(0.0209,-0.0744704599711237,0.003));
#31977=CARTESIAN_POINT('',(0.0209,-0.03005,0.0024));
#31978=CARTESIAN_POINT('Origin',(0.02090000000001,-0.03005,0.00300000000001001));
#31979=CARTESIAN_POINT('',(0.0209,-0.02924999999999,0.0024));
#31980=CARTESIAN_POINT('',(0.0209,-0.0744704599711237,0.0024));
#31981=CARTESIAN_POINT('Origin',(0.02090000000001,-0.02924999999999,0.00300000000001001));
#31982=CARTESIAN_POINT('Origin',(0.0209,-0.0744704599711237,0.001));
#31983=CARTESIAN_POINT('',(0.0209,-0.03005,0.000400000000000001));
#31984=CARTESIAN_POINT('Origin',(0.02090000000001,-0.03005,0.00100000000001));
#31985=CARTESIAN_POINT('',(0.0209,-0.02924999999999,0.000400000000000001));
#31986=CARTESIAN_POINT('',(0.0209,-0.0744704599711237,0.0004));
#31987=CARTESIAN_POINT('Origin',(0.02090000000001,-0.02924999999999,0.00100000000001));
#31988=CARTESIAN_POINT('Origin',(0.0209,-0.0744704599711237,-0.003));
#31989=CARTESIAN_POINT('',(0.0209,-0.03005,-0.0036));
#31990=CARTESIAN_POINT('Origin',(0.02090000000001,-0.03005,-0.00300000000001));
#31991=CARTESIAN_POINT('',(0.0209,-0.02924999999999,-0.0036));
#31992=CARTESIAN_POINT('',(0.0209,-0.0744704599711237,-0.0036));
#31993=CARTESIAN_POINT('Origin',(0.02090000000001,-0.02924999999999,-0.00300000000001));
#31994=CARTESIAN_POINT('Origin',(0.0209,-0.0744704599711237,-0.005));
#31995=CARTESIAN_POINT('',(0.0209,-0.03005,-0.0056));
#31996=CARTESIAN_POINT('Origin',(0.02090000000001,-0.03005,-0.00500000000001));
#31997=CARTESIAN_POINT('',(0.0209,-0.02924999999999,-0.0056));
#31998=CARTESIAN_POINT('',(0.0209,-0.0744704599711237,-0.0056));
#31999=CARTESIAN_POINT('Origin',(0.02090000000001,-0.02924999999999,-0.00500000000001));
#32000=CARTESIAN_POINT('Origin',(0.0209,-0.0744704599711237,-0.001));
#32001=CARTESIAN_POINT('',(0.0209,-0.03005,-0.0016));
#32002=CARTESIAN_POINT('Origin',(0.02090000000001,-0.03005,-0.00100000000001));
#32003=CARTESIAN_POINT('',(0.0209,-0.02924999999999,-0.0016));
#32004=CARTESIAN_POINT('',(0.0209,-0.0744704599711237,-0.0016));
#32005=CARTESIAN_POINT('Origin',(0.02090000000001,-0.02924999999999,-0.00100000000001));
#32006=CARTESIAN_POINT('Origin',(0.0199,-0.03005,0.0071));
#32007=CARTESIAN_POINT('',(0.0199,-0.03005,0.0071));
#32008=CARTESIAN_POINT('',(0.0079000000000001,-0.03005,0.019));
#32009=CARTESIAN_POINT('',(0.0199000000000101,-0.03005,0.00710000000001001));
#32010=CARTESIAN_POINT('',(0.0199,-0.02925,0.0071));
#32011=CARTESIAN_POINT('',(0.0199000000000101,-0.03005,0.00710000000001001));
#32012=CARTESIAN_POINT('',(0.0079000000000001,-0.02925,0.019));
#32013=CARTESIAN_POINT('',(0.0199000000000101,-0.02924999999999,0.00710000000001001));
#32014=CARTESIAN_POINT('',(0.00790000000001011,-0.03005,0.0190000000000101));
#32015=CARTESIAN_POINT('Origin',(0.0264,-0.03005,0.0071));
#32016=CARTESIAN_POINT('',(0.0264,-0.03005,0.0071));
#32017=CARTESIAN_POINT('',(0.0264000000000101,-0.03005,0.00710000000000998));
#32018=CARTESIAN_POINT('',(0.0264,-0.02925,0.0071));
#32019=CARTESIAN_POINT('',(0.0264000000000101,-0.03005,0.00710000000000998));
#32020=CARTESIAN_POINT('',(0.0264000000000101,-0.02924999999999,0.00710000000000998));
#32021=CARTESIAN_POINT('Origin',(0.0019000000000001,-0.03005,0.019));
#32022=CARTESIAN_POINT('',(0.0019000000000001,-0.03005,0.019));
#32023=CARTESIAN_POINT('',(0.00190000000000008,-0.03005,0.0136930639376293));
#32024=CARTESIAN_POINT('',(0.00190000000001011,-0.03005,0.0190000000000101));
#32025=CARTESIAN_POINT('',(0.0019000000000001,-0.02925,0.019));
#32026=CARTESIAN_POINT('',(0.00190000000001011,-0.03005,0.0190000000000101));
#32027=CARTESIAN_POINT('',(0.00190000000000008,-0.02925,0.0136930639376293));
#32028=CARTESIAN_POINT('',(0.00190000000001011,-0.02924999999999,0.0190000000000101));
#32029=CARTESIAN_POINT('',(0.00190000000001009,-0.03005,0.0136930639376393));
#32030=CARTESIAN_POINT('Origin',(0.0079000000000001,-0.03005,0.019));
#32031=CARTESIAN_POINT('',(0.00790000000001011,-0.03005,0.0190000000000101));
#32032=CARTESIAN_POINT('',(0.00790000000001011,-0.02924999999999,0.0190000000000101));
#32033=CARTESIAN_POINT('Origin',(0.0199,-0.03005,-0.0071));
#32034=CARTESIAN_POINT('',(0.0199,-0.03005,-0.0071));
#32035=CARTESIAN_POINT('',(0.0079,-0.03005,-0.019));
#32036=CARTESIAN_POINT('',(0.01990000000001,-0.03005,-0.00710000000000999));
#32037=CARTESIAN_POINT('',(0.0079,-0.02925,-0.019));
#32038=CARTESIAN_POINT('',(0.00790000000000993,-0.03005,-0.0190000000000099));
#32039=CARTESIAN_POINT('',(0.0199,-0.02925,-0.0071));
#32040=CARTESIAN_POINT('',(0.01990000000001,-0.02924999999999,-0.00710000000000999));
#32041=CARTESIAN_POINT('',(0.01990000000001,-0.03005,-0.00710000000000999));
#32042=CARTESIAN_POINT('Origin',(0.0264,-0.03005,-0.0071));
#32043=CARTESIAN_POINT('',(0.0264,-0.03005,-0.0071));
#32044=CARTESIAN_POINT('',(0.02640000000001,-0.03005,-0.00710000000001002));
#32045=CARTESIAN_POINT('',(0.0264,-0.02925,-0.0071));
#32046=CARTESIAN_POINT('',(0.02640000000001,-0.02924999999999,-0.00710000000001002));
#32047=CARTESIAN_POINT('',(0.02640000000001,-0.03005,-0.00710000000001002));
#32048=CARTESIAN_POINT('Origin',(0.0264,-0.03005,-2.31739922485765E-17));
#32049=CARTESIAN_POINT('',(0.02640000000001,-0.03005,-1.00231739922486E-14));
#32050=CARTESIAN_POINT('',(0.02640000000001,-0.02924999999999,-1.00231669383767E-14));
#32051=CARTESIAN_POINT('Origin',(0.000650000000000017,-0.03005,9.37463700322586E-17));
#32052=CARTESIAN_POINT('',(0.00189999999999995,-0.03005,-0.0136930639376291));
#32053=CARTESIAN_POINT('Origin',(0.000650000000000017,-0.03005,9.37463700322586E-17));
#32054=CARTESIAN_POINT('',(0.00189999999999995,-0.02925,-0.0136930639376291));
#32055=CARTESIAN_POINT('Origin',(0.000650000000000017,-0.02924999999999,
9.37534239041485E-17));
#32056=CARTESIAN_POINT('',(0.00190000000000995,-0.03005,-0.0136930639376391));
#32057=CARTESIAN_POINT('Origin',(0.00189999999999993,-0.03005,-0.019));
#32058=CARTESIAN_POINT('',(0.00189999999999993,-0.03005,-0.019));
#32059=CARTESIAN_POINT('',(0.00190000000000993,-0.03005,-0.0190000000000099));
#32060=CARTESIAN_POINT('',(0.00189999999999993,-0.02925,-0.019));
#32061=CARTESIAN_POINT('',(0.00190000000000993,-0.02924999999999,-0.0190000000000099));
#32062=CARTESIAN_POINT('',(0.00190000000000993,-0.03005,-0.0190000000000099));
#32063=CARTESIAN_POINT('Origin',(0.0079,-0.03005,-0.019));
#32064=CARTESIAN_POINT('',(0.00790000000000993,-0.03005,-0.0190000000000099));
#32065=CARTESIAN_POINT('',(0.00790000000000993,-0.02924999999999,-0.0190000000000099));
#32066=CARTESIAN_POINT('Origin',(0.01415,-0.02925,-0.0095));
#32067=CARTESIAN_POINT('Origin',(0.01415,-0.03005,-0.0095));
#34823=UNCERTAINTY_MEASURE_WITH_UNIT(LENGTH_MEASURE(1.E-5),#34877,
'DISTANCE_ACCURACY_VALUE',
'Maximum model space distance between geometric entities at asserted c
onnectivities');
#34841=UNCERTAINTY_MEASURE_WITH_UNIT(LENGTH_MEASURE(1.E-5),#34877,
'DISTANCE_ACCURACY_VALUE',
'Maximum model space distance between geometric entities at asserted c
onnectivities');
#34858=(
GEOMETRIC_REPRESENTATION_CONTEXT(3)
GLOBAL_UNCERTAINTY_ASSIGNED_CONTEXT((#34823))
GLOBAL_UNIT_ASSIGNED_CONTEXT((#34877,#34878,#34879))
REPRESENTATION_CONTEXT('','3D')
);
#34876=(
GEOMETRIC_REPRESENTATION_CONTEXT(3)
GLOBAL_UNCERTAINTY_ASSIGNED_CONTEXT((#34841))
GLOBAL_UNIT_ASSIGNED_CONTEXT((#34877,#34878,#34879))
REPRESENTATION_CONTEXT('','3D')
);
#34877=(
LENGTH_UNIT()
NAMED_UNIT(*)
SI_UNIT($,.METRE.)
);
#34878=(
NAMED_UNIT(*)
PLANE_ANGLE_UNIT()
SI_UNIT($,.RADIAN.)
);
#34879=(
NAMED_UNIT(*)
SI_UNIT($,.STERADIAN.)
SOLID_ANGLE_UNIT()
);
#34896=SHAPE_DEFINITION_REPRESENTATION(#34930,#35000);
#34930=PRODUCT_DEFINITION_SHAPE('',$,#35035);
#35000=SHAPE_REPRESENTATION('',(#21215),#34858);
#35018=PRODUCT_DEFINITION_CONTEXT('part definition',#35122,'design');
#35035=PRODUCT_DEFINITION('Motor PCB','Motor PCB',#35069,#35018);
#35069=PRODUCT_DEFINITION_FORMATION('',$,#35140);
#35122=APPLICATION_CONTEXT('Managed model based 3d engineering');
#35123=PRODUCT_CONTEXT('part definition',#35122,'mechanical');
#35140=PRODUCT('Motor PCB','Motor PCB',
'LEGAL AND USAGE DISCLAIMER: this Data/Model is provided \X2\201C\X0\A
S IS\X2\201D\X0\ for informational and representational only. It is a 
geometric approximation and is NOT engineered, certified, or guarantee
d for dimensional accuracy, exact tolerances, or production-level prec
ision. Vendor disclaims all implied warranties including fitness for a
 particular purpose. DO NOT USE FOR DIRECT PHYSICAL MANUFACTURING, AUT
OMATED PRODUCTION, OR SAFETY-CRITICAL SYSTEMS without independent engi
neering verification and resolution of any design discrepancies.',(#35123));
#35161=PRESENTATION_STYLE_ASSIGNMENT((#35170));
#35170=SURFACE_STYLE_USAGE(.BOTH.,#35179);
#35179=SURFACE_SIDE_STYLE('',(#35188));
#35188=SURFACE_STYLE_FILL_AREA(#35197);
#35197=FILL_AREA_STYLE('Aluminum - Anodized Glossy (Blue)',(#35206));
#35206=FILL_AREA_STYLE_COLOUR('Aluminum - Anodized Glossy (Blue)',#35215);
#35215=COLOUR_RGB('Aluminum - Anodized Glossy (Blue)',0.349019607843137,
0.584313725490196,0.854901960784314);
ENDSEC;
END-ISO-10303-21;
